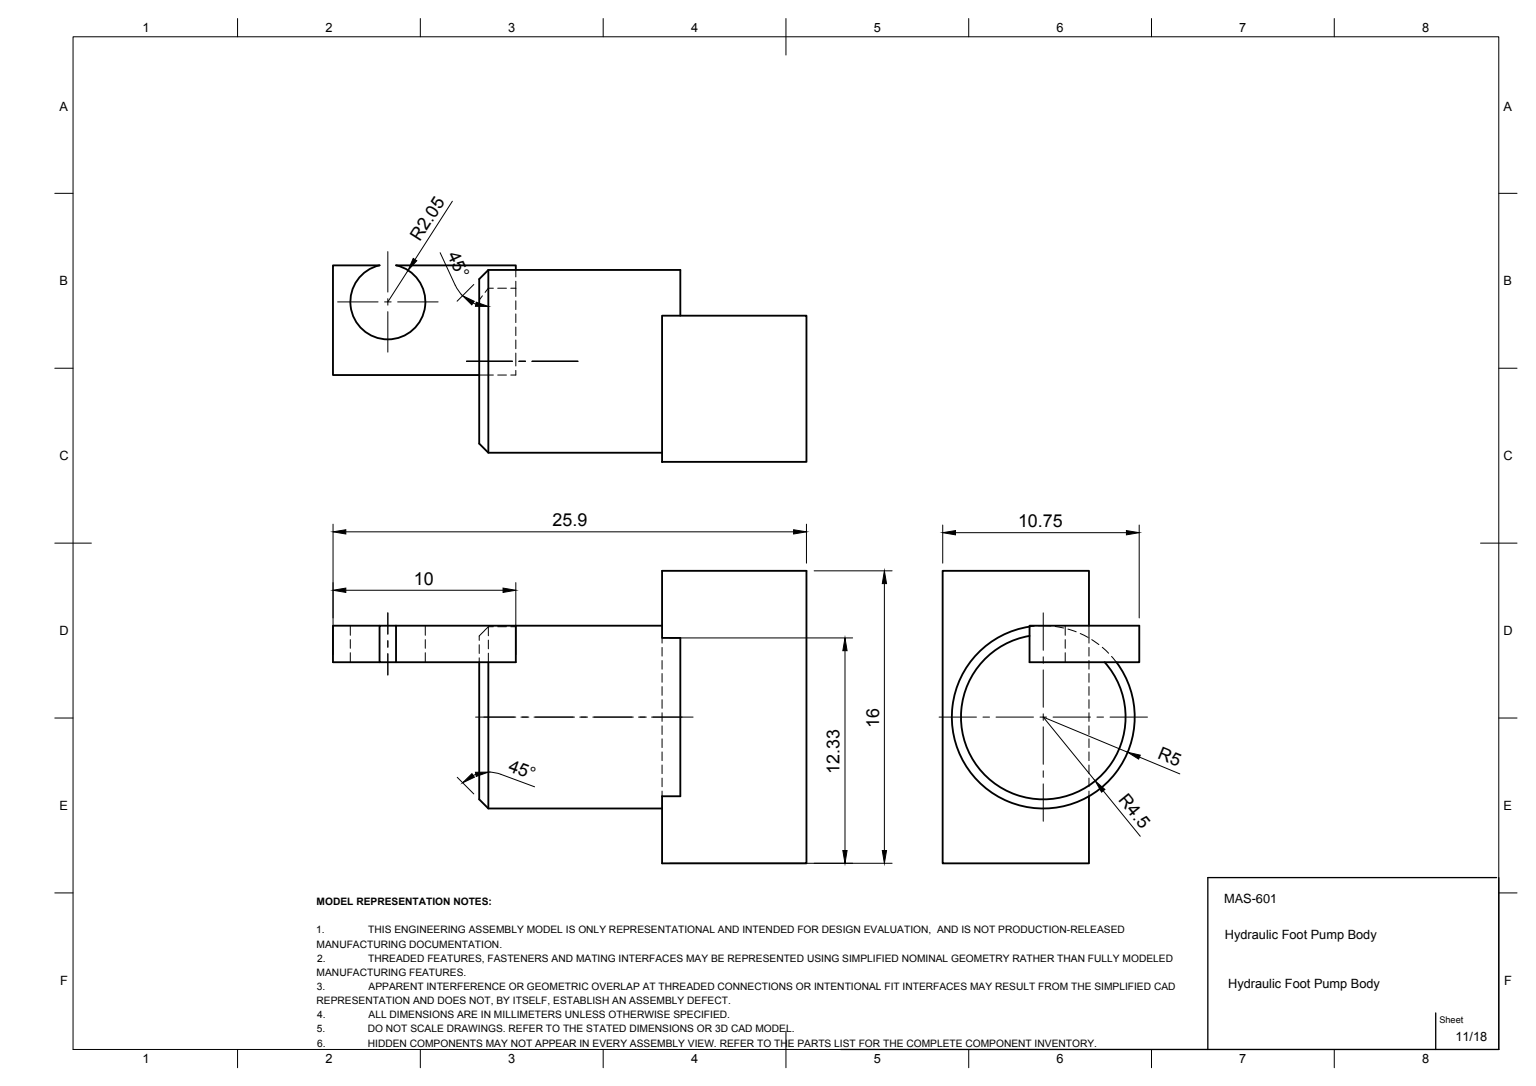
ISO-10303-21;
HEADER;
FILE_DESCRIPTION((''),'2;1');
FILE_NAME('Hydraulic Foot Pump Body.step','2026-10-06T07:37:42+05:00',(''),(''),'','','');
FILE_SCHEMA (('AUTOMOTIVE_DESIGN { 1 0 10303 214 3 1 1 }'));
ENDSEC;
DATA;
#10=MECHANICAL_DESIGN_GEOMETRIC_PRESENTATION_REPRESENTATION('',(#379),#18757);
#245=(
BOUNDED_CURVE()
B_SPLINE_CURVE(2,(#14772,#14773,#14774),.UNSPECIFIED.,.F.,.F.)
B_SPLINE_CURVE_WITH_KNOTS((3,3),(0.,0.0816843221416426),.UNSPECIFIED.)
CURVE()
GEOMETRIC_REPRESENTATION_ITEM()
RATIONAL_B_SPLINE_CURVE((1.,1.00231931413628,1.))
REPRESENTATION_ITEM('')
) ;
#246=(
BOUNDED_CURVE()
B_SPLINE_CURVE(2,(#14806,#14807,#14808),.UNSPECIFIED.,.F.,.F.)
B_SPLINE_CURVE_WITH_KNOTS((3,3),(0.,0.0711625451007686),.UNSPECIFIED.)
CURVE()
GEOMETRIC_REPRESENTATION_ITEM()
RATIONAL_B_SPLINE_CURVE((1.,1.00142359213772,1.))
REPRESENTATION_ITEM('')
) ;
#345=SHAPE_REPRESENTATION_RELATIONSHIP('SRR','None',#18863,#362) ;
#362=ADVANCED_BREP_SHAPE_REPRESENTATION('',(#396),#18746) ;
#379=STYLED_ITEM('',(#18957),#396) ;
#396=MANIFOLD_SOLID_BREP('Hydraulic Foot Pump Body',#9548) ;
#574=CYLINDRICAL_SURFACE('',#10123,2.05) ;
#575=CYLINDRICAL_SURFACE('',#10143,5.) ;
#868=PLANE('',#10126) ;
#869=PLANE('',#10127) ;
#870=PLANE('',#10128) ;
#871=PLANE('',#10129) ;
#872=PLANE('',#10131) ;
#873=PLANE('',#10133) ;
#874=PLANE('',#10134) ;
#875=PLANE('',#10135) ;
#876=PLANE('',#10136) ;
#877=PLANE('',#10141) ;
#878=PLANE('',#10146) ;
#879=PLANE('',#10147) ;
#880=PLANE('',#10148) ;
#881=PLANE('',#10149) ;
#882=PLANE('',#10150) ;
#883=PLANE('',#10151) ;
#1290=FACE_OUTER_BOUND('',#1878,.T.) ;
#1291=FACE_OUTER_BOUND('',#1879,.T.) ;
#1292=FACE_OUTER_BOUND('',#1880,.T.) ;
#1293=FACE_OUTER_BOUND('',#1881,.T.) ;
#1294=FACE_OUTER_BOUND('',#1882,.T.) ;
#1295=FACE_OUTER_BOUND('',#1883,.T.) ;
#1296=FACE_OUTER_BOUND('',#1884,.T.) ;
#1297=FACE_OUTER_BOUND('',#1885,.T.) ;
#1298=FACE_OUTER_BOUND('',#1886,.T.) ;
#1299=FACE_OUTER_BOUND('',#1887,.T.) ;
#1300=FACE_OUTER_BOUND('',#1888,.T.) ;
#1301=FACE_OUTER_BOUND('',#1889,.T.) ;
#1302=FACE_OUTER_BOUND('',#1890,.T.) ;
#1303=FACE_OUTER_BOUND('',#1891,.T.) ;
#1304=FACE_OUTER_BOUND('',#1892,.T.) ;
#1305=FACE_OUTER_BOUND('',#1893,.T.) ;
#1306=FACE_OUTER_BOUND('',#1894,.T.) ;
#1307=FACE_OUTER_BOUND('',#1895,.T.) ;
#1308=FACE_OUTER_BOUND('',#1896,.T.) ;
#1878=EDGE_LOOP('',(#7351,#7352,#7353,#7354)) ;
#1879=EDGE_LOOP('',(#7355,#7356,#7357,#7358,#7359,#7360,#7361,#7362,#7363)) ;
#1880=EDGE_LOOP('',(#7364,#7365,#7366,#7367)) ;
#1881=EDGE_LOOP('',(#7368,#7369,#7370,#7371)) ;
#1882=EDGE_LOOP('',(#7372,#7373,#7374)) ;
#1883=EDGE_LOOP('',(#7375,#7376,#7377,#7378)) ;
#1884=EDGE_LOOP('',(#7379,#7380,#7381,#7382,#7383,#7384,#7385)) ;
#1885=EDGE_LOOP('',(#7386,#7387,#7388,#7389)) ;
#1886=EDGE_LOOP('',(#7390,#7391,#7392,#7393,#7394,#7395,#7396)) ;
#1887=EDGE_LOOP('',(#7397,#7398,#7399)) ;
#1888=EDGE_LOOP('',(#7400,#7401,#7402,#7403,#7404)) ;
#1889=EDGE_LOOP('',(#7405,#7406)) ;
#1890=EDGE_LOOP('',(#7407,#7408,#7409,#7410,#7411,#7412,#7413,#7414,#7415,
#7416,#7417,#7418,#7419)) ;
#1891=EDGE_LOOP('',(#7420,#7421,#7422,#7423,#7424,#7425,#7426)) ;
#1892=EDGE_LOOP('',(#7427,#7428,#7429,#7430)) ;
#1893=EDGE_LOOP('',(#7431,#7432,#7433,#7434,#7435,#7436,#7437,#7438)) ;
#1894=EDGE_LOOP('',(#7439,#7440,#7441,#7442)) ;
#1895=EDGE_LOOP('',(#7443,#7444,#7445,#7446)) ;
#1896=EDGE_LOOP('',(#7447,#7448,#7449,#7450)) ;
#2551=LINE('',#14756,#3322) ;
#2552=LINE('',#14760,#3323) ;
#2553=LINE('',#14764,#3324) ;
#2554=LINE('',#14766,#3325) ;
#2555=LINE('',#14768,#3326) ;
#2556=LINE('',#14770,#3327) ;
#2557=LINE('',#14776,#3328) ;
#2558=LINE('',#14778,#3329) ;
#2559=LINE('',#14779,#3330) ;
#2560=LINE('',#14782,#3331) ;
#2561=LINE('',#14783,#3332) ;
#2562=LINE('',#14786,#3333) ;
#2563=LINE('',#14787,#3334) ;
#2564=LINE('',#14793,#3335) ;
#2565=LINE('',#14794,#3336) ;
#2566=LINE('',#14797,#3337) ;
#2567=LINE('',#14800,#3338) ;
#2568=LINE('',#14802,#3339) ;
#2569=LINE('',#14803,#3340) ;
#2570=LINE('',#14805,#3341) ;
#2571=LINE('',#14810,#3342) ;
#2572=LINE('',#14821,#3343) ;
#2573=LINE('',#14825,#3344) ;
#2574=LINE('',#14828,#3345) ;
#2575=LINE('',#14830,#3346) ;
#2576=LINE('',#14834,#3347) ;
#2577=LINE('',#14836,#3348) ;
#2578=LINE('',#14838,#3349) ;
#2579=LINE('',#14840,#3350) ;
#2580=LINE('',#14841,#3351) ;
#2581=LINE('',#14845,#3352) ;
#2582=LINE('',#14846,#3353) ;
#2583=LINE('',#14847,#3354) ;
#2584=LINE('',#14850,#3355) ;
#2585=LINE('',#14851,#3356) ;
#2586=LINE('',#14854,#3357) ;
#2587=LINE('',#14855,#3358) ;
#2588=LINE('',#14857,#3359) ;
#3322=VECTOR('',#11787,10.) ;
#3323=VECTOR('',#11790,10.) ;
#3324=VECTOR('',#11795,10.) ;
#3325=VECTOR('',#11796,10.) ;
#3326=VECTOR('',#11797,10.) ;
#3327=VECTOR('',#11798,10.) ;
#3328=VECTOR('',#11799,10.) ;
#3329=VECTOR('',#11800,10.) ;
#3330=VECTOR('',#11801,10.) ;
#3331=VECTOR('',#11804,10.) ;
#3332=VECTOR('',#11805,10.) ;
#3333=VECTOR('',#11808,10.) ;
#3334=VECTOR('',#11809,10.) ;
#3335=VECTOR('',#11814,10.) ;
#3336=VECTOR('',#11815,10.) ;
#3337=VECTOR('',#11820,10.) ;
#3338=VECTOR('',#11823,10.) ;
#3339=VECTOR('',#11824,10.) ;
#3340=VECTOR('',#11825,10.) ;
#3341=VECTOR('',#11826,10.) ;
#3342=VECTOR('',#11829,10.) ;
#3343=VECTOR('',#11844,10.) ;
#3344=VECTOR('',#11849,5.) ;
#3345=VECTOR('',#11852,10.) ;
#3346=VECTOR('',#11853,10.) ;
#3347=VECTOR('',#11858,10.) ;
#3348=VECTOR('',#11859,10.) ;
#3349=VECTOR('',#11860,10.) ;
#3350=VECTOR('',#11861,10.) ;
#3351=VECTOR('',#11862,10.) ;
#3352=VECTOR('',#11865,10.) ;
#3353=VECTOR('',#11866,10.) ;
#3354=VECTOR('',#11867,10.) ;
#3355=VECTOR('',#11870,10.) ;
#3356=VECTOR('',#11871,10.) ;
#3357=VECTOR('',#11874,10.) ;
#3358=VECTOR('',#11875,10.) ;
#3359=VECTOR('',#11878,10.) ;
#3940=CIRCLE('',#10124,2.05) ;
#3941=CIRCLE('',#10125,2.05) ;
#3942=CIRCLE('',#10130,5.) ;
#3943=CIRCLE('',#10132,5.) ;
#3944=CIRCLE('',#10137,4.49999999999999) ;
#3945=CIRCLE('',#10139,5.) ;
#3946=CIRCLE('',#10140,5.) ;
#3947=CIRCLE('',#10142,5.) ;
#3948=CIRCLE('',#10144,5.) ;
#3949=CIRCLE('',#10145,5.) ;
#4480=VERTEX_POINT('',#14754) ;
#4481=VERTEX_POINT('',#14755) ;
#4482=VERTEX_POINT('',#14757) ;
#4483=VERTEX_POINT('',#14759) ;
#4484=VERTEX_POINT('',#14763) ;
#4485=VERTEX_POINT('',#14765) ;
#4486=VERTEX_POINT('',#14767) ;
#4487=VERTEX_POINT('',#14769) ;
#4488=VERTEX_POINT('',#14771) ;
#4489=VERTEX_POINT('',#14775) ;
#4490=VERTEX_POINT('',#14777) ;
#4491=VERTEX_POINT('',#14781) ;
#4492=VERTEX_POINT('',#14785) ;
#4493=VERTEX_POINT('',#14789) ;
#4494=VERTEX_POINT('',#14790) ;
#4495=VERTEX_POINT('',#14792) ;
#4496=VERTEX_POINT('',#14799) ;
#4497=VERTEX_POINT('',#14801) ;
#4498=VERTEX_POINT('',#14804) ;
#4499=VERTEX_POINT('',#14815) ;
#4500=VERTEX_POINT('',#14819) ;
#4501=VERTEX_POINT('',#14820) ;
#4502=VERTEX_POINT('',#14824) ;
#4503=VERTEX_POINT('',#14826) ;
#4504=VERTEX_POINT('',#14829) ;
#4505=VERTEX_POINT('',#14833) ;
#4506=VERTEX_POINT('',#14835) ;
#4507=VERTEX_POINT('',#14837) ;
#4508=VERTEX_POINT('',#14839) ;
#4509=VERTEX_POINT('',#14843) ;
#4510=VERTEX_POINT('',#14844) ;
#4511=VERTEX_POINT('',#14849) ;
#4512=VERTEX_POINT('',#14853) ;
#5522=EDGE_CURVE('',#4480,#4481,#2551,.T.) ;
#5523=EDGE_CURVE('',#4482,#4480,#3940,.T.) ;
#5524=EDGE_CURVE('',#4483,#4482,#2552,.T.) ;
#5525=EDGE_CURVE('',#4481,#4483,#3941,.T.) ;
#5526=EDGE_CURVE('',#4480,#4484,#2553,.T.) ;
#5527=EDGE_CURVE('',#4484,#4485,#2554,.T.) ;
#5528=EDGE_CURVE('',#4485,#4486,#2555,.T.) ;
#5529=EDGE_CURVE('',#4487,#4486,#2556,.T.) ;
#5530=EDGE_CURVE('',#4488,#4487,#245,.T.) ;
#5531=EDGE_CURVE('',#4489,#4488,#2557,.T.) ;
#5532=EDGE_CURVE('',#4489,#4490,#2558,.T.) ;
#5533=EDGE_CURVE('',#4490,#4482,#2559,.T.) ;
#5534=EDGE_CURVE('',#4491,#4481,#2560,.T.) ;
#5535=EDGE_CURVE('',#4484,#4491,#2561,.T.) ;
#5536=EDGE_CURVE('',#4490,#4492,#2562,.T.) ;
#5537=EDGE_CURVE('',#4483,#4492,#2563,.T.) ;
#5538=EDGE_CURVE('',#4493,#4494,#3942,.T.) ;
#5539=EDGE_CURVE('',#4493,#4495,#2564,.T.) ;
#5540=EDGE_CURVE('',#4494,#4495,#2565,.T.) ;
#5541=EDGE_CURVE('',#4494,#4489,#3943,.T.) ;
#5542=EDGE_CURVE('',#4492,#4494,#2566,.T.) ;
#5543=EDGE_CURVE('',#4486,#4496,#2567,.T.) ;
#5544=EDGE_CURVE('',#4485,#4497,#2568,.T.) ;
#5545=EDGE_CURVE('',#4495,#4497,#2569,.T.) ;
#5546=EDGE_CURVE('',#4498,#4493,#2570,.T.) ;
#5547=EDGE_CURVE('',#4496,#4498,#246,.T.) ;
#5548=EDGE_CURVE('',#4497,#4491,#2571,.T.) ;
#5549=EDGE_CURVE('',#4496,#4487,#3944,.T.) ;
#5550=EDGE_CURVE('',#4498,#4499,#3945,.T.) ;
#5551=EDGE_CURVE('',#4499,#4488,#3946,.T.) ;
#5552=EDGE_CURVE('',#4500,#4501,#2572,.T.) ;
#5553=EDGE_CURVE('',#4501,#4500,#3947,.T.) ;
#5554=EDGE_CURVE('',#4499,#4502,#2573,.T.) ;
#5555=EDGE_CURVE('',#4503,#4502,#3948,.T.) ;
#5556=EDGE_CURVE('',#4501,#4503,#2574,.T.) ;
#5557=EDGE_CURVE('',#4504,#4500,#2575,.T.) ;
#5558=EDGE_CURVE('',#4502,#4504,#3949,.T.) ;
#5559=EDGE_CURVE('',#4504,#4505,#2576,.T.) ;
#5560=EDGE_CURVE('',#4505,#4506,#2577,.T.) ;
#5561=EDGE_CURVE('',#4506,#4507,#2578,.T.) ;
#5562=EDGE_CURVE('',#4507,#4508,#2579,.T.) ;
#5563=EDGE_CURVE('',#4508,#4503,#2580,.T.) ;
#5564=EDGE_CURVE('',#4509,#4510,#2581,.T.) ;
#5565=EDGE_CURVE('',#4510,#4506,#2582,.T.) ;
#5566=EDGE_CURVE('',#4509,#4505,#2583,.T.) ;
#5567=EDGE_CURVE('',#4511,#4508,#2584,.T.) ;
#5568=EDGE_CURVE('',#4511,#4509,#2585,.T.) ;
#5569=EDGE_CURVE('',#4512,#4511,#2586,.T.) ;
#5570=EDGE_CURVE('',#4512,#4507,#2587,.T.) ;
#5571=EDGE_CURVE('',#4510,#4512,#2588,.T.) ;
#7351=ORIENTED_EDGE('',*,*,#5522,.F.) ;
#7352=ORIENTED_EDGE('',*,*,#5523,.F.) ;
#7353=ORIENTED_EDGE('',*,*,#5524,.F.) ;
#7354=ORIENTED_EDGE('',*,*,#5525,.F.) ;
#7355=ORIENTED_EDGE('',*,*,#5523,.T.) ;
#7356=ORIENTED_EDGE('',*,*,#5526,.T.) ;
#7357=ORIENTED_EDGE('',*,*,#5527,.T.) ;
#7358=ORIENTED_EDGE('',*,*,#5528,.T.) ;
#7359=ORIENTED_EDGE('',*,*,#5529,.F.) ;
#7360=ORIENTED_EDGE('',*,*,#5530,.F.) ;
#7361=ORIENTED_EDGE('',*,*,#5531,.F.) ;
#7362=ORIENTED_EDGE('',*,*,#5532,.T.) ;
#7363=ORIENTED_EDGE('',*,*,#5533,.T.) ;
#7364=ORIENTED_EDGE('',*,*,#5522,.T.) ;
#7365=ORIENTED_EDGE('',*,*,#5534,.F.) ;
#7366=ORIENTED_EDGE('',*,*,#5535,.F.) ;
#7367=ORIENTED_EDGE('',*,*,#5526,.F.) ;
#7368=ORIENTED_EDGE('',*,*,#5524,.T.) ;
#7369=ORIENTED_EDGE('',*,*,#5533,.F.) ;
#7370=ORIENTED_EDGE('',*,*,#5536,.T.) ;
#7371=ORIENTED_EDGE('',*,*,#5537,.F.) ;
#7372=ORIENTED_EDGE('',*,*,#5538,.F.) ;
#7373=ORIENTED_EDGE('',*,*,#5539,.T.) ;
#7374=ORIENTED_EDGE('',*,*,#5540,.F.) ;
#7375=ORIENTED_EDGE('',*,*,#5541,.F.) ;
#7376=ORIENTED_EDGE('',*,*,#5542,.F.) ;
#7377=ORIENTED_EDGE('',*,*,#5536,.F.) ;
#7378=ORIENTED_EDGE('',*,*,#5532,.F.) ;
#7379=ORIENTED_EDGE('',*,*,#5543,.F.) ;
#7380=ORIENTED_EDGE('',*,*,#5528,.F.) ;
#7381=ORIENTED_EDGE('',*,*,#5544,.T.) ;
#7382=ORIENTED_EDGE('',*,*,#5545,.F.) ;
#7383=ORIENTED_EDGE('',*,*,#5539,.F.) ;
#7384=ORIENTED_EDGE('',*,*,#5546,.F.) ;
#7385=ORIENTED_EDGE('',*,*,#5547,.F.) ;
#7386=ORIENTED_EDGE('',*,*,#5527,.F.) ;
#7387=ORIENTED_EDGE('',*,*,#5535,.T.) ;
#7388=ORIENTED_EDGE('',*,*,#5548,.F.) ;
#7389=ORIENTED_EDGE('',*,*,#5544,.F.) ;
#7390=ORIENTED_EDGE('',*,*,#5525,.T.) ;
#7391=ORIENTED_EDGE('',*,*,#5537,.T.) ;
#7392=ORIENTED_EDGE('',*,*,#5542,.T.) ;
#7393=ORIENTED_EDGE('',*,*,#5540,.T.) ;
#7394=ORIENTED_EDGE('',*,*,#5545,.T.) ;
#7395=ORIENTED_EDGE('',*,*,#5548,.T.) ;
#7396=ORIENTED_EDGE('',*,*,#5534,.T.) ;
#7397=ORIENTED_EDGE('',*,*,#5529,.T.) ;
#7398=ORIENTED_EDGE('',*,*,#5543,.T.) ;
#7399=ORIENTED_EDGE('',*,*,#5549,.T.) ;
#7400=ORIENTED_EDGE('',*,*,#5530,.T.) ;
#7401=ORIENTED_EDGE('',*,*,#5549,.F.) ;
#7402=ORIENTED_EDGE('',*,*,#5547,.T.) ;
#7403=ORIENTED_EDGE('',*,*,#5550,.T.) ;
#7404=ORIENTED_EDGE('',*,*,#5551,.T.) ;
#7405=ORIENTED_EDGE('',*,*,#5552,.F.) ;
#7406=ORIENTED_EDGE('',*,*,#5553,.F.) ;
#7407=ORIENTED_EDGE('',*,*,#5531,.T.) ;
#7408=ORIENTED_EDGE('',*,*,#5551,.F.) ;
#7409=ORIENTED_EDGE('',*,*,#5554,.T.) ;
#7410=ORIENTED_EDGE('',*,*,#5555,.F.) ;
#7411=ORIENTED_EDGE('',*,*,#5556,.F.) ;
#7412=ORIENTED_EDGE('',*,*,#5553,.T.) ;
#7413=ORIENTED_EDGE('',*,*,#5557,.F.) ;
#7414=ORIENTED_EDGE('',*,*,#5558,.F.) ;
#7415=ORIENTED_EDGE('',*,*,#5554,.F.) ;
#7416=ORIENTED_EDGE('',*,*,#5550,.F.) ;
#7417=ORIENTED_EDGE('',*,*,#5546,.T.) ;
#7418=ORIENTED_EDGE('',*,*,#5538,.T.) ;
#7419=ORIENTED_EDGE('',*,*,#5541,.T.) ;
#7420=ORIENTED_EDGE('',*,*,#5555,.T.) ;
#7421=ORIENTED_EDGE('',*,*,#5558,.T.) ;
#7422=ORIENTED_EDGE('',*,*,#5559,.T.) ;
#7423=ORIENTED_EDGE('',*,*,#5560,.T.) ;
#7424=ORIENTED_EDGE('',*,*,#5561,.T.) ;
#7425=ORIENTED_EDGE('',*,*,#5562,.T.) ;
#7426=ORIENTED_EDGE('',*,*,#5563,.T.) ;
#7427=ORIENTED_EDGE('',*,*,#5564,.T.) ;
#7428=ORIENTED_EDGE('',*,*,#5565,.T.) ;
#7429=ORIENTED_EDGE('',*,*,#5560,.F.) ;
#7430=ORIENTED_EDGE('',*,*,#5566,.F.) ;
#7431=ORIENTED_EDGE('',*,*,#5556,.T.) ;
#7432=ORIENTED_EDGE('',*,*,#5563,.F.) ;
#7433=ORIENTED_EDGE('',*,*,#5567,.F.) ;
#7434=ORIENTED_EDGE('',*,*,#5568,.T.) ;
#7435=ORIENTED_EDGE('',*,*,#5566,.T.) ;
#7436=ORIENTED_EDGE('',*,*,#5559,.F.) ;
#7437=ORIENTED_EDGE('',*,*,#5557,.T.) ;
#7438=ORIENTED_EDGE('',*,*,#5552,.T.) ;
#7439=ORIENTED_EDGE('',*,*,#5569,.T.) ;
#7440=ORIENTED_EDGE('',*,*,#5567,.T.) ;
#7441=ORIENTED_EDGE('',*,*,#5562,.F.) ;
#7442=ORIENTED_EDGE('',*,*,#5570,.F.) ;
#7443=ORIENTED_EDGE('',*,*,#5571,.T.) ;
#7444=ORIENTED_EDGE('',*,*,#5570,.T.) ;
#7445=ORIENTED_EDGE('',*,*,#5561,.F.) ;
#7446=ORIENTED_EDGE('',*,*,#5565,.F.) ;
#7447=ORIENTED_EDGE('',*,*,#5571,.F.) ;
#7448=ORIENTED_EDGE('',*,*,#5564,.F.) ;
#7449=ORIENTED_EDGE('',*,*,#5568,.F.) ;
#7450=ORIENTED_EDGE('',*,*,#5569,.F.) ;
#9009=CONICAL_SURFACE('',#10138,4.75,0.785398163397457) ;
#9226=ADVANCED_FACE('',(#1290),#574,.F.) ;
#9227=ADVANCED_FACE('',(#1291),#868,.F.) ;
#9228=ADVANCED_FACE('',(#1292),#869,.T.) ;
#9229=ADVANCED_FACE('',(#1293),#870,.T.) ;
#9230=ADVANCED_FACE('',(#1294),#871,.T.) ;
#9231=ADVANCED_FACE('',(#1295),#872,.T.) ;
#9232=ADVANCED_FACE('',(#1296),#873,.T.) ;
#9233=ADVANCED_FACE('',(#1297),#874,.T.) ;
#9234=ADVANCED_FACE('',(#1298),#875,.T.) ;
#9235=ADVANCED_FACE('',(#1299),#876,.T.) ;
#9236=ADVANCED_FACE('',(#1300),#9009,.T.) ;
#9237=ADVANCED_FACE('',(#1301),#877,.T.) ;
#9238=ADVANCED_FACE('',(#1302),#575,.T.) ;
#9239=ADVANCED_FACE('',(#1303),#878,.T.) ;
#9240=ADVANCED_FACE('',(#1304),#879,.T.) ;
#9241=ADVANCED_FACE('',(#1305),#880,.T.) ;
#9242=ADVANCED_FACE('',(#1306),#881,.T.) ;
#9243=ADVANCED_FACE('',(#1307),#882,.T.) ;
#9244=ADVANCED_FACE('',(#1308),#883,.F.) ;
#9548=CLOSED_SHELL('',(#9226,#9227,#9228,#9229,#9230,#9231,#9232,#9233,
#9234,#9235,#9236,#9237,#9238,#9239,#9240,#9241,#9242,#9243,#9244)) ;
#10122=AXIS2_PLACEMENT_3D('',#14752,#11783,#11784) ;
#10123=AXIS2_PLACEMENT_3D('',#14753,#11785,#11786) ;
#10124=AXIS2_PLACEMENT_3D('',#14758,#11788,#11789) ;
#10125=AXIS2_PLACEMENT_3D('',#14761,#11791,#11792) ;
#10126=AXIS2_PLACEMENT_3D('',#14762,#11793,#11794) ;
#10127=AXIS2_PLACEMENT_3D('',#14780,#11802,#11803) ;
#10128=AXIS2_PLACEMENT_3D('',#14784,#11806,#11807) ;
#10129=AXIS2_PLACEMENT_3D('',#14788,#11810,#11811) ;
#10130=AXIS2_PLACEMENT_3D('',#14791,#11812,#11813) ;
#10131=AXIS2_PLACEMENT_3D('',#14795,#11816,#11817) ;
#10132=AXIS2_PLACEMENT_3D('',#14796,#11818,#11819) ;
#10133=AXIS2_PLACEMENT_3D('',#14798,#11821,#11822) ;
#10134=AXIS2_PLACEMENT_3D('',#14809,#11827,#11828) ;
#10135=AXIS2_PLACEMENT_3D('',#14811,#11830,#11831) ;
#10136=AXIS2_PLACEMENT_3D('',#14812,#11832,#11833) ;
#10137=AXIS2_PLACEMENT_3D('',#14813,#11834,#11835) ;
#10138=AXIS2_PLACEMENT_3D('',#14814,#11836,#11837) ;
#10139=AXIS2_PLACEMENT_3D('',#14816,#11838,#11839) ;
#10140=AXIS2_PLACEMENT_3D('',#14817,#11840,#11841) ;
#10141=AXIS2_PLACEMENT_3D('',#14818,#11842,#11843) ;
#10142=AXIS2_PLACEMENT_3D('',#14822,#11845,#11846) ;
#10143=AXIS2_PLACEMENT_3D('',#14823,#11847,#11848) ;
#10144=AXIS2_PLACEMENT_3D('',#14827,#11850,#11851) ;
#10145=AXIS2_PLACEMENT_3D('',#14831,#11854,#11855) ;
#10146=AXIS2_PLACEMENT_3D('',#14832,#11856,#11857) ;
#10147=AXIS2_PLACEMENT_3D('',#14842,#11863,#11864) ;
#10148=AXIS2_PLACEMENT_3D('',#14848,#11868,#11869) ;
#10149=AXIS2_PLACEMENT_3D('',#14852,#11872,#11873) ;
#10150=AXIS2_PLACEMENT_3D('',#14856,#11876,#11877) ;
#10151=AXIS2_PLACEMENT_3D('',#14858,#11879,#11880) ;
#11783=DIRECTION('axis',(0.,0.,1.)) ;
#11784=DIRECTION('refdir',(1.,0.,0.)) ;
#11785=DIRECTION('center_axis',(0.,1.,0.)) ;
#11786=DIRECTION('ref_axis',(-1.,0.,1.22464679914735E-16)) ;
#11787=DIRECTION('',(0.,1.,0.)) ;
#11788=DIRECTION('center_axis',(0.,1.,0.)) ;
#11789=DIRECTION('ref_axis',(1.,0.,0.)) ;
#11790=DIRECTION('',(0.,-1.,0.)) ;
#11791=DIRECTION('center_axis',(0.,-1.,0.)) ;
#11792=DIRECTION('ref_axis',(1.,0.,0.)) ;
#11793=DIRECTION('center_axis',(0.,1.,0.)) ;
#11794=DIRECTION('ref_axis',(1.,0.,0.)) ;
#11795=DIRECTION('',(0.,0.,1.)) ;
#11796=DIRECTION('',(-1.,0.,0.)) ;
#11797=DIRECTION('',(0.,0.,-1.)) ;
#11798=DIRECTION('',(-1.,0.,0.)) ;
#11799=DIRECTION('',(0.,0.,1.)) ;
#11800=DIRECTION('',(1.,0.,0.)) ;
#11801=DIRECTION('',(0.,0.,1.)) ;
#11802=DIRECTION('center_axis',(1.,0.,0.)) ;
#11803=DIRECTION('ref_axis',(0.,0.,-1.)) ;
#11804=DIRECTION('',(0.,0.,-1.)) ;
#11805=DIRECTION('',(0.,1.,0.)) ;
#11806=DIRECTION('center_axis',(1.,0.,0.)) ;
#11807=DIRECTION('ref_axis',(0.,0.,-1.)) ;
#11808=DIRECTION('',(0.,1.,0.)) ;
#11809=DIRECTION('',(0.,0.,-1.)) ;
#11810=DIRECTION('center_axis',(0.,0.,-1.)) ;
#11811=DIRECTION('ref_axis',(-1.,0.,0.)) ;
#11812=DIRECTION('center_axis',(0.,0.,-1.)) ;
#11813=DIRECTION('ref_axis',(1.,0.,0.)) ;
#11814=DIRECTION('',(0.,1.,0.)) ;
#11815=DIRECTION('',(-1.,0.,0.)) ;
#11816=DIRECTION('center_axis',(0.,0.,-1.)) ;
#11817=DIRECTION('ref_axis',(-1.,0.,0.)) ;
#11818=DIRECTION('center_axis',(0.,0.,-1.)) ;
#11819=DIRECTION('ref_axis',(1.,0.,0.)) ;
#11820=DIRECTION('',(-1.,0.,0.)) ;
#11821=DIRECTION('center_axis',(-1.,0.,0.)) ;
#11822=DIRECTION('ref_axis',(0.,0.,1.)) ;
#11823=DIRECTION('',(0.,1.,0.)) ;
#11824=DIRECTION('',(0.,1.,0.)) ;
#11825=DIRECTION('',(0.,0.,1.)) ;
#11826=DIRECTION('',(0.,0.,-1.)) ;
#11827=DIRECTION('center_axis',(0.,0.,1.)) ;
#11828=DIRECTION('ref_axis',(1.,0.,0.)) ;
#11829=DIRECTION('',(1.,0.,0.)) ;
#11830=DIRECTION('center_axis',(0.,1.,0.)) ;
#11831=DIRECTION('ref_axis',(0.,0.,1.)) ;
#11832=DIRECTION('center_axis',(0.,0.,1.)) ;
#11833=DIRECTION('ref_axis',(1.,0.,0.)) ;
#11834=DIRECTION('center_axis',(0.,0.,1.)) ;
#11835=DIRECTION('ref_axis',(1.,0.,0.)) ;
#11836=DIRECTION('center_axis',(0.,0.,-1.)) ;
#11837=DIRECTION('ref_axis',(-0.338432122698804,-0.940990806716825,0.)) ;
#11838=DIRECTION('center_axis',(0.,0.,1.)) ;
#11839=DIRECTION('ref_axis',(1.,0.,0.)) ;
#11840=DIRECTION('center_axis',(0.,0.,1.)) ;
#11841=DIRECTION('ref_axis',(1.,0.,0.)) ;
#11842=DIRECTION('center_axis',(0.,0.,-1.)) ;
#11843=DIRECTION('ref_axis',(-1.,0.,0.)) ;
#11844=DIRECTION('',(0.,-1.,0.)) ;
#11845=DIRECTION('center_axis',(0.,0.,1.)) ;
#11846=DIRECTION('ref_axis',(1.,0.,0.)) ;
#11847=DIRECTION('center_axis',(0.,0.,1.)) ;
#11848=DIRECTION('ref_axis',(1.,0.,0.)) ;
#11849=DIRECTION('',(0.,0.,-1.)) ;
#11850=DIRECTION('center_axis',(0.,0.,-1.)) ;
#11851=DIRECTION('ref_axis',(1.,0.,0.)) ;
#11852=DIRECTION('',(0.,0.,1.)) ;
#11853=DIRECTION('',(0.,0.,-1.)) ;
#11854=DIRECTION('center_axis',(0.,0.,-1.)) ;
#11855=DIRECTION('ref_axis',(1.,0.,0.)) ;
#11856=DIRECTION('center_axis',(0.,0.,1.)) ;
#11857=DIRECTION('ref_axis',(1.,0.,0.)) ;
#11858=DIRECTION('',(0.,1.,0.)) ;
#11859=DIRECTION('',(-1.,0.,0.)) ;
#11860=DIRECTION('',(0.,-1.,0.)) ;
#11861=DIRECTION('',(1.,0.,0.)) ;
#11862=DIRECTION('',(0.,1.,0.)) ;
#11863=DIRECTION('center_axis',(0.,1.,0.)) ;
#11864=DIRECTION('ref_axis',(-1.,0.,0.)) ;
#11865=DIRECTION('',(-1.,0.,0.)) ;
#11866=DIRECTION('',(0.,0.,1.)) ;
#11867=DIRECTION('',(0.,0.,1.)) ;
#11868=DIRECTION('center_axis',(1.,0.,0.)) ;
#11869=DIRECTION('ref_axis',(0.,1.,0.)) ;
#11870=DIRECTION('',(0.,0.,1.)) ;
#11871=DIRECTION('',(0.,1.,0.)) ;
#11872=DIRECTION('center_axis',(0.,-1.,0.)) ;
#11873=DIRECTION('ref_axis',(1.,0.,0.)) ;
#11874=DIRECTION('',(1.,0.,0.)) ;
#11875=DIRECTION('',(0.,0.,1.)) ;
#11876=DIRECTION('center_axis',(-1.,0.,0.)) ;
#11877=DIRECTION('ref_axis',(0.,-1.,0.)) ;
#11878=DIRECTION('',(0.,-1.,0.)) ;
#11879=DIRECTION('center_axis',(0.,0.,1.)) ;
#11880=DIRECTION('ref_axis',(1.,0.,0.)) ;
#14752=CARTESIAN_POINT('',(0.,0.,0.)) ;
#14753=CARTESIAN_POINT('Origin',(96.,2.5,52.)) ;
#14754=CARTESIAN_POINT('',(98.,3.,52.45)) ;
#14755=CARTESIAN_POINT('',(98.,5.,52.45)) ;
#14756=CARTESIAN_POINT('',(98.,2.5,52.45)) ;
#14757=CARTESIAN_POINT('',(98.,3.,51.55)) ;
#14758=CARTESIAN_POINT('Origin',(96.,3.,52.)) ;
#14759=CARTESIAN_POINT('',(98.,5.,51.55)) ;
#14760=CARTESIAN_POINT('',(98.,2.5,51.55)) ;
#14761=CARTESIAN_POINT('Origin',(96.,5.,52.)) ;
#14762=CARTESIAN_POINT('Origin',(95.,3.,50.)) ;
#14763=CARTESIAN_POINT('',(98.,3.,55.)) ;
#14764=CARTESIAN_POINT('',(98.,3.,45.)) ;
#14765=CARTESIAN_POINT('',(92.,3.,55.)) ;
#14766=CARTESIAN_POINT('',(98.,3.,55.)) ;
#14767=CARTESIAN_POINT('',(92.,3.,47.)) ;
#14768=CARTESIAN_POINT('',(92.,3.,55.)) ;
#14769=CARTESIAN_POINT('',(96.1041019662497,3.,47.)) ;
#14770=CARTESIAN_POINT('',(93.875,3.,47.)) ;
#14771=CARTESIAN_POINT('',(96.75,3.,46.5)) ;
#14772=CARTESIAN_POINT('Ctrl Pts',(96.75,3.,46.5)) ;
#14773=CARTESIAN_POINT('Ctrl Pts',(96.4100536664472,3.,46.7719570668423)) ;
#14774=CARTESIAN_POINT('Ctrl Pts',(96.1041019662497,3.,47.)) ;
#14775=CARTESIAN_POINT('',(96.75,3.,45.)) ;
#14776=CARTESIAN_POINT('',(96.75,3.,41.25)) ;
#14777=CARTESIAN_POINT('',(98.,3.,45.)) ;
#14778=CARTESIAN_POINT('',(92.,3.,45.)) ;
#14779=CARTESIAN_POINT('',(98.,3.,45.)) ;
#14780=CARTESIAN_POINT('Origin',(98.,3.,55.)) ;
#14781=CARTESIAN_POINT('',(98.,5.,55.)) ;
#14782=CARTESIAN_POINT('',(98.,5.,45.)) ;
#14783=CARTESIAN_POINT('',(98.,3.,55.)) ;
#14784=CARTESIAN_POINT('Origin',(98.,3.,55.)) ;
#14785=CARTESIAN_POINT('',(98.,5.,45.)) ;
#14786=CARTESIAN_POINT('',(98.,3.,45.)) ;
#14787=CARTESIAN_POINT('',(98.,5.,45.)) ;
#14788=CARTESIAN_POINT('Origin',(98.,3.,45.)) ;
#14789=CARTESIAN_POINT('',(92.,4.9434299833213,45.)) ;
#14790=CARTESIAN_POINT('',(92.75,5.,45.)) ;
#14791=CARTESIAN_POINT('Origin',(92.75,0.,45.)) ;
#14792=CARTESIAN_POINT('',(92.,5.,45.)) ;
#14793=CARTESIAN_POINT('',(92.,3.,45.)) ;
#14794=CARTESIAN_POINT('',(92.,5.,45.)) ;
#14795=CARTESIAN_POINT('Origin',(98.,3.,45.)) ;
#14796=CARTESIAN_POINT('Origin',(92.75,0.,45.)) ;
#14797=CARTESIAN_POINT('',(92.,5.,45.)) ;
#14798=CARTESIAN_POINT('Origin',(92.,3.,45.)) ;
#14799=CARTESIAN_POINT('',(92.,4.4370598373247,47.)) ;
#14800=CARTESIAN_POINT('',(92.,1.5,47.)) ;
#14801=CARTESIAN_POINT('',(92.,5.,55.)) ;
#14802=CARTESIAN_POINT('',(92.,3.,55.)) ;
#14803=CARTESIAN_POINT('',(92.,5.,55.)) ;
#14804=CARTESIAN_POINT('',(92.,4.9434299833213,46.5)) ;
#14805=CARTESIAN_POINT('',(92.,4.9434299833213,41.25)) ;
#14806=CARTESIAN_POINT('Ctrl Pts',(92.,4.43705983732471,47.)) ;
#14807=CARTESIAN_POINT('Ctrl Pts',(92.,4.67691938017707,46.7634953012913)) ;
#14808=CARTESIAN_POINT('Ctrl Pts',(92.,4.9434299833213,46.5)) ;
#14809=CARTESIAN_POINT('Origin',(92.,3.,55.)) ;
#14810=CARTESIAN_POINT('',(98.,5.,55.)) ;
#14811=CARTESIAN_POINT('Origin',(95.,5.,50.)) ;
#14812=CARTESIAN_POINT('Origin',(92.75,0.,47.)) ;
#14813=CARTESIAN_POINT('Origin',(92.75,0.,47.)) ;
#14814=CARTESIAN_POINT('Origin',(92.75,0.,46.75)) ;
#14815=CARTESIAN_POINT('',(87.75,-6.12323399573677E-16,46.5)) ;
#14816=CARTESIAN_POINT('Origin',(92.75,0.,46.5)) ;
#14817=CARTESIAN_POINT('Origin',(92.75,0.,46.5)) ;
#14818=CARTESIAN_POINT('Origin',(97.75,0.,36.)) ;
#14819=CARTESIAN_POINT('',(95.25,4.33012701892219,36.)) ;
#14820=CARTESIAN_POINT('',(95.25,-4.33012701892219,36.)) ;
#14821=CARTESIAN_POINT('',(95.25,-4.,36.)) ;
#14822=CARTESIAN_POINT('Origin',(92.75,0.,36.)) ;
#14823=CARTESIAN_POINT('Origin',(92.75,0.,41.25)) ;
#14824=CARTESIAN_POINT('',(87.75,-6.12323399573677E-16,37.)) ;
#14825=CARTESIAN_POINT('',(87.75,-6.12323399573677E-16,41.25)) ;
#14826=CARTESIAN_POINT('',(95.25,-4.33012701892219,37.)) ;
#14827=CARTESIAN_POINT('Origin',(92.75,0.,37.)) ;
#14828=CARTESIAN_POINT('',(95.25,-4.33012701892219,41.25)) ;
#14829=CARTESIAN_POINT('',(95.25,4.33012701892219,37.)) ;
#14830=CARTESIAN_POINT('',(95.25,4.33012701892219,41.25)) ;
#14831=CARTESIAN_POINT('Origin',(92.75,0.,37.)) ;
#14832=CARTESIAN_POINT('Origin',(91.25,0.,37.)) ;
#14833=CARTESIAN_POINT('',(95.25,8.,37.)) ;
#14834=CARTESIAN_POINT('',(95.25,-8.,37.)) ;
#14835=CARTESIAN_POINT('',(87.25,8.,37.)) ;
#14836=CARTESIAN_POINT('',(95.25,8.,37.)) ;
#14837=CARTESIAN_POINT('',(87.25,-8.,37.)) ;
#14838=CARTESIAN_POINT('',(87.25,8.,37.)) ;
#14839=CARTESIAN_POINT('',(95.25,-8.,37.)) ;
#14840=CARTESIAN_POINT('',(87.25,-8.,37.)) ;
#14841=CARTESIAN_POINT('',(95.25,-8.,37.)) ;
#14842=CARTESIAN_POINT('Origin',(95.25,8.,29.1)) ;
#14843=CARTESIAN_POINT('',(95.25,8.,29.1)) ;
#14844=CARTESIAN_POINT('',(87.25,8.,29.1)) ;
#14845=CARTESIAN_POINT('',(95.25,8.,29.1)) ;
#14846=CARTESIAN_POINT('',(87.25,8.,29.1)) ;
#14847=CARTESIAN_POINT('',(95.25,8.,29.1)) ;
#14848=CARTESIAN_POINT('Origin',(95.25,-8.,29.1)) ;
#14849=CARTESIAN_POINT('',(95.25,-8.,29.1)) ;
#14850=CARTESIAN_POINT('',(95.25,-8.,29.1)) ;
#14851=CARTESIAN_POINT('',(95.25,-8.,29.1)) ;
#14852=CARTESIAN_POINT('Origin',(87.25,-8.,29.1)) ;
#14853=CARTESIAN_POINT('',(87.25,-8.,29.1)) ;
#14854=CARTESIAN_POINT('',(87.25,-8.,29.1)) ;
#14855=CARTESIAN_POINT('',(87.25,-8.,29.1)) ;
#14856=CARTESIAN_POINT('Origin',(87.25,8.,29.1)) ;
#14857=CARTESIAN_POINT('',(87.25,8.,29.1)) ;
#14858=CARTESIAN_POINT('Origin',(91.25,0.,29.1)) ;
#18727=UNCERTAINTY_MEASURE_WITH_UNIT(LENGTH_MEASURE(0.01),#18758,
'DISTANCE_ACCURACY_VALUE',
'Maximum model space distance between geometric entities at asserted c
onnectivities') ;
#18738=UNCERTAINTY_MEASURE_WITH_UNIT(LENGTH_MEASURE(0.01),#18758,
'DISTANCE_ACCURACY_VALUE',
'Maximum model space distance between geometric entities at asserted c
onnectivities') ;
#18746=(
GEOMETRIC_REPRESENTATION_CONTEXT(3)
GLOBAL_UNCERTAINTY_ASSIGNED_CONTEXT((#18727))
GLOBAL_UNIT_ASSIGNED_CONTEXT((#18758,#18760,#18761))
REPRESENTATION_CONTEXT('','3D')
) ;
#18757=(
GEOMETRIC_REPRESENTATION_CONTEXT(3)
GLOBAL_UNCERTAINTY_ASSIGNED_CONTEXT((#18738))
GLOBAL_UNIT_ASSIGNED_CONTEXT((#18758,#18760,#18761))
REPRESENTATION_CONTEXT('','3D')
) ;
#18758=(
LENGTH_UNIT()
NAMED_UNIT(*)
SI_UNIT(.MILLI.,.METRE.)
) ;
#18760=(
NAMED_UNIT(*)
PLANE_ANGLE_UNIT()
SI_UNIT($,.RADIAN.)
) ;
#18761=(
NAMED_UNIT(*)
SI_UNIT($,.STERADIAN.)
SOLID_ANGLE_UNIT()
) ;
#18769=SHAPE_DEFINITION_REPRESENTATION(#18787,#18863) ;
#18787=PRODUCT_DEFINITION_SHAPE('',$,#18882) ;
#18863=SHAPE_REPRESENTATION('',(#10122),#18746) ;
#18874=PRODUCT_DEFINITION_CONTEXT('part definition',#18930,'design') ;
#18882=PRODUCT_DEFINITION('Hydraulic Foot Pump Body',
'Hydraulic Foot Pump Body',#18900,#18874) ;
#18900=PRODUCT_DEFINITION_FORMATION('',$,#18939) ;
#18930=APPLICATION_CONTEXT(
'Core Data for Automotive Mechanical Design Process') ;
#18931=PRODUCT_CONTEXT('part definition',#18930,'mechanical') ;
#18939=PRODUCT('Hydraulic Foot Pump Body','Hydraulic Foot Pump Body',$,(#18931)) ;
#18957=PRESENTATION_STYLE_ASSIGNMENT((#18975)) ;
#18975=SURFACE_STYLE_USAGE(.BOTH.,#18993) ;
#18993=SURFACE_SIDE_STYLE('',(#19011)) ;
#19011=SURFACE_STYLE_FILL_AREA(#19029) ;
#19029=FILL_AREA_STYLE(
'MAS-253 Metallic Sheet - Hydraulic Foot Pump Body',(#19047)) ;
#19047=FILL_AREA_STYLE_COLOUR(
'MAS-253 Metallic Sheet - Hydraulic Foot Pump Body',#19065) ;
#19065=COLOUR_RGB('MAS-253 Metallic Sheet - Hydraulic Foot Pump Body', 0.66274510, 0.83137255, 0.94901961) ;
ENDSEC;
END-ISO-10303-21;
